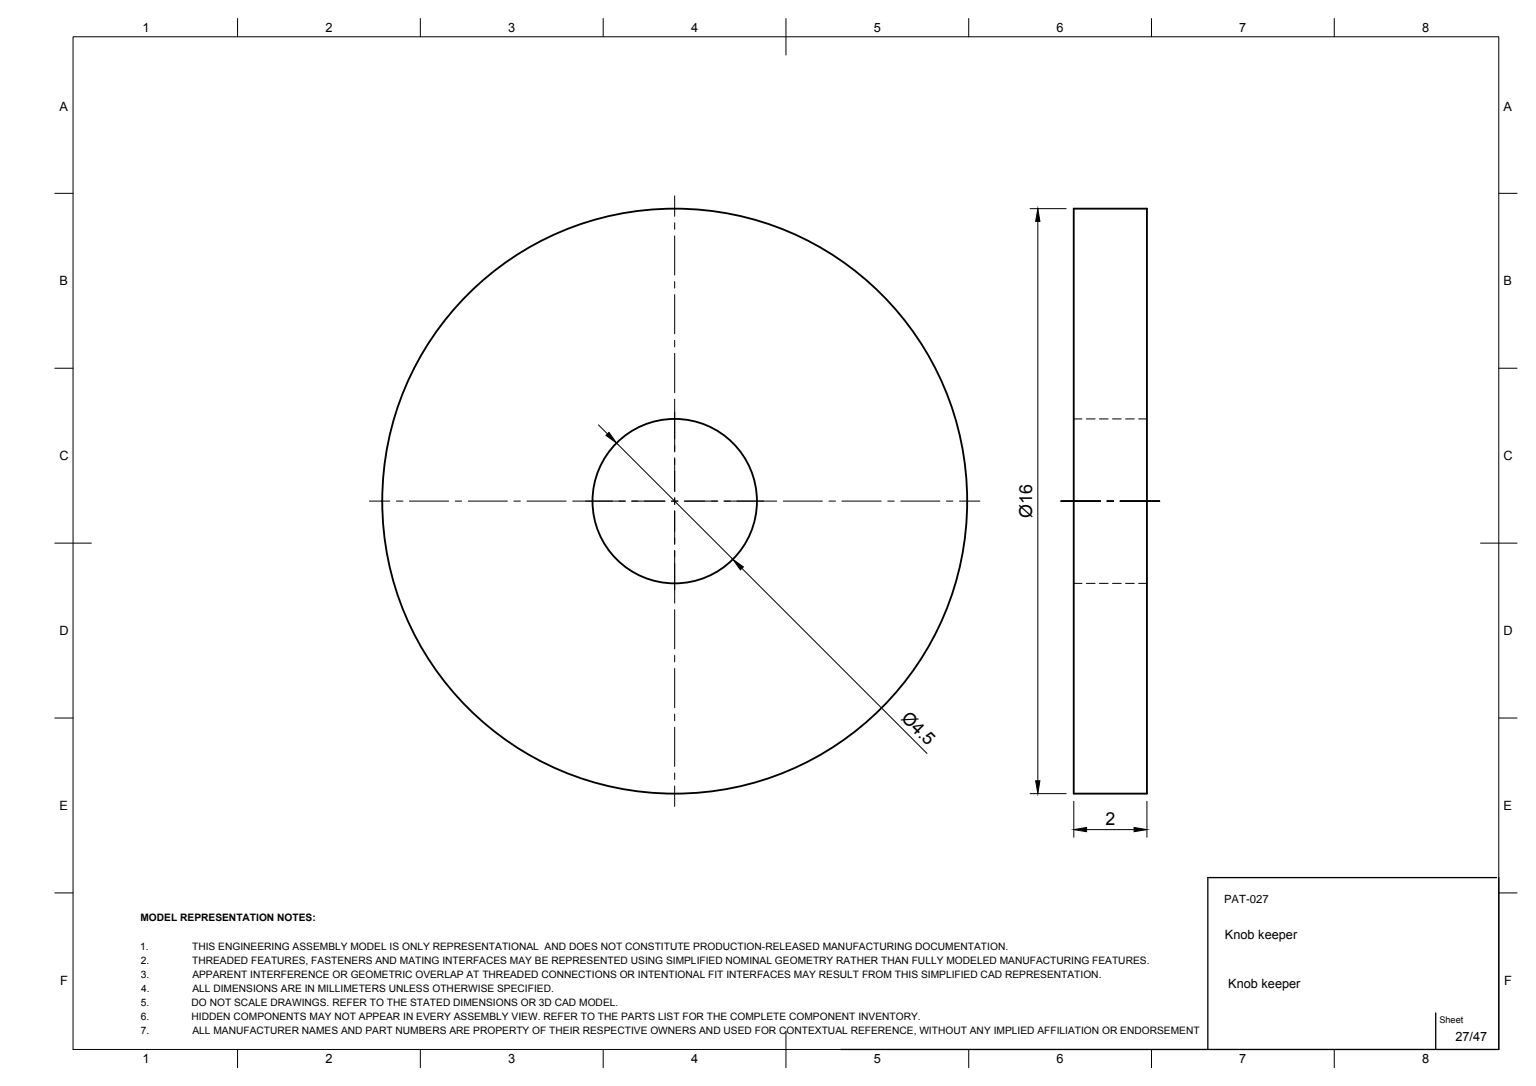
ISO-10303-21;
HEADER;
/* Generated by software containing ST-Developer
 * from STEP Tools, Inc. (www.steptools.com) 
 */

FILE_DESCRIPTION(
/* description */ ('Crank-driven oscillating fan base (mechanism only)'),

/* implementation_level */ '2;1');

FILE_NAME(
/* name */ 'Knob keeper.step',
/* time_stamp */ '2026-10-28T03:25:00-07:00',
/* author */ (''),
/* organization */ (''),
/* preprocessor_version */ 'ST-DEVELOPER v20.2',
/* originating_system */ 'Autodesk Translation Framework v15.17.0.0',
/* authorisation */ '');

FILE_SCHEMA (('AUTOMOTIVE_DESIGN { 1 0 10303 214 3 1 1 }'));
ENDSEC;

DATA;
#10=MECHANICAL_DESIGN_GEOMETRIC_PRESENTATION_REPRESENTATION('',(#464),#11916);
#376=SHAPE_REPRESENTATION_RELATIONSHIP('SRR','None',#12102,#416);
#416=ADVANCED_BREP_SHAPE_REPRESENTATION('',(#511),#11893);
#464=STYLED_ITEM('',(#12361),#511);
#511=MANIFOLD_SOLID_BREP('Body1',#6095);
#634=FACE_BOUND('',#1580,.T.);
#635=FACE_BOUND('',#1582,.T.);
#790=PLANE('',#7047);
#791=PLANE('',#7048);
#1098=FACE_OUTER_BOUND('',#1577,.T.);
#1099=FACE_OUTER_BOUND('',#1578,.T.);
#1100=FACE_OUTER_BOUND('',#1579,.T.);
#1101=FACE_OUTER_BOUND('',#1581,.T.);
#1577=EDGE_LOOP('',(#4958,#4959,#4960,#4961));
#1578=EDGE_LOOP('',(#4962,#4963,#4964,#4965));
#1579=EDGE_LOOP('',(#4966));
#1580=EDGE_LOOP('',(#4967));
#1581=EDGE_LOOP('',(#4968));
#1582=EDGE_LOOP('',(#4969));
#1966=LINE('',#11033,#2299);
#1967=LINE('',#11039,#2300);
#2299=VECTOR('',#8547,0.225);
#2300=VECTOR('',#8554,0.8);
#2705=CIRCLE('',#7042,0.225);
#2706=CIRCLE('',#7043,0.225);
#2707=CIRCLE('',#7045,0.8);
#2708=CIRCLE('',#7046,0.8);
#3136=VERTEX_POINT('',#11030);
#3137=VERTEX_POINT('',#11032);
#3138=VERTEX_POINT('',#11036);
#3139=VERTEX_POINT('',#11038);
#3774=EDGE_CURVE('',#3136,#3136,#2705,.T.);
#3775=EDGE_CURVE('',#3136,#3137,#1966,.T.);
#3776=EDGE_CURVE('',#3137,#3137,#2706,.T.);
#3777=EDGE_CURVE('',#3138,#3138,#2707,.T.);
#3778=EDGE_CURVE('',#3138,#3139,#1967,.T.);
#3779=EDGE_CURVE('',#3139,#3139,#2708,.T.);
#4958=ORIENTED_EDGE('',*,*,#3774,.F.);
#4959=ORIENTED_EDGE('',*,*,#3775,.T.);
#4960=ORIENTED_EDGE('',*,*,#3776,.T.);
#4961=ORIENTED_EDGE('',*,*,#3775,.F.);
#4962=ORIENTED_EDGE('',*,*,#3777,.F.);
#4963=ORIENTED_EDGE('',*,*,#3778,.T.);
#4964=ORIENTED_EDGE('',*,*,#3779,.T.);
#4965=ORIENTED_EDGE('',*,*,#3778,.F.);
#4966=ORIENTED_EDGE('',*,*,#3777,.T.);
#4967=ORIENTED_EDGE('',*,*,#3774,.T.);
#4968=ORIENTED_EDGE('',*,*,#3779,.F.);
#4969=ORIENTED_EDGE('',*,*,#3776,.F.);
#5635=CYLINDRICAL_SURFACE('',#7041,0.225);
#5636=CYLINDRICAL_SURFACE('',#7044,0.8);
#5904=ADVANCED_FACE('',(#1098),#5635,.F.);
#5905=ADVANCED_FACE('',(#1099),#5636,.T.);
#5906=ADVANCED_FACE('',(#1100,#634),#790,.T.);
#5907=ADVANCED_FACE('',(#1101,#635),#791,.F.);
#6095=CLOSED_SHELL('',(#5904,#5905,#5906,#5907));
#7040=AXIS2_PLACEMENT_3D('',#11028,#8541,#8542);
#7041=AXIS2_PLACEMENT_3D('',#11029,#8543,#8544);
#7042=AXIS2_PLACEMENT_3D('',#11031,#8545,#8546);
#7043=AXIS2_PLACEMENT_3D('',#11034,#8548,#8549);
#7044=AXIS2_PLACEMENT_3D('',#11035,#8550,#8551);
#7045=AXIS2_PLACEMENT_3D('',#11037,#8552,#8553);
#7046=AXIS2_PLACEMENT_3D('',#11040,#8555,#8556);
#7047=AXIS2_PLACEMENT_3D('',#11041,#8557,#8558);
#7048=AXIS2_PLACEMENT_3D('',#11042,#8559,#8560);
#8541=DIRECTION('axis',(0.,0.,1.));
#8542=DIRECTION('refdir',(1.,0.,0.));
#8543=DIRECTION('center_axis',(0.,0.,1.));
#8544=DIRECTION('ref_axis',(1.,0.,0.));
#8545=DIRECTION('center_axis',(0.,0.,-1.));
#8546=DIRECTION('ref_axis',(1.,0.,0.));
#8547=DIRECTION('',(0.,0.,-1.));
#8548=DIRECTION('center_axis',(0.,0.,-1.));
#8549=DIRECTION('ref_axis',(1.,0.,0.));
#8550=DIRECTION('center_axis',(0.,0.,1.));
#8551=DIRECTION('ref_axis',(1.,0.,0.));
#8552=DIRECTION('center_axis',(0.,0.,1.));
#8553=DIRECTION('ref_axis',(1.,0.,0.));
#8554=DIRECTION('',(0.,0.,-1.));
#8555=DIRECTION('center_axis',(0.,0.,1.));
#8556=DIRECTION('ref_axis',(1.,0.,0.));
#8557=DIRECTION('center_axis',(0.,0.,1.));
#8558=DIRECTION('ref_axis',(1.,0.,0.));
#8559=DIRECTION('center_axis',(0.,0.,1.));
#8560=DIRECTION('ref_axis',(1.,0.,0.));
#11028=CARTESIAN_POINT('',(0.,0.,0.));
#11029=CARTESIAN_POINT('Origin',(0.,0.,8.));
#11030=CARTESIAN_POINT('',(-0.225,-2.75545529808154E-17,8.2));
#11031=CARTESIAN_POINT('Origin',(0.,0.,8.2));
#11032=CARTESIAN_POINT('',(-0.225,-2.75545529808154E-17,8.));
#11033=CARTESIAN_POINT('',(-0.225,-2.75545529808154E-17,8.));
#11034=CARTESIAN_POINT('Origin',(0.,0.,8.));
#11035=CARTESIAN_POINT('Origin',(0.,0.,8.));
#11036=CARTESIAN_POINT('',(-0.8,-9.79717439317883E-17,8.2));
#11037=CARTESIAN_POINT('Origin',(0.,0.,8.2));
#11038=CARTESIAN_POINT('',(-0.8,-9.79717439317883E-17,8.));
#11039=CARTESIAN_POINT('',(-0.8,-9.79717439317883E-17,8.));
#11040=CARTESIAN_POINT('Origin',(0.,0.,8.));
#11041=CARTESIAN_POINT('Origin',(0.,0.,8.2));
#11042=CARTESIAN_POINT('Origin',(0.,0.,8.));
#11846=UNCERTAINTY_MEASURE_WITH_UNIT(LENGTH_MEASURE(0.001),#11917,
'DISTANCE_ACCURACY_VALUE',
'Maximum model space distance between geometric entities at asserted c
onnectivities');
#11869=UNCERTAINTY_MEASURE_WITH_UNIT(LENGTH_MEASURE(0.001),#11917,
'DISTANCE_ACCURACY_VALUE',
'Maximum model space distance between geometric entities at asserted c
onnectivities');
#11893=(
GEOMETRIC_REPRESENTATION_CONTEXT(3)
GLOBAL_UNCERTAINTY_ASSIGNED_CONTEXT((#11846))
GLOBAL_UNIT_ASSIGNED_CONTEXT((#11917,#11919,#11920))
REPRESENTATION_CONTEXT('','3D')
);
#11916=(
GEOMETRIC_REPRESENTATION_CONTEXT(3)
GLOBAL_UNCERTAINTY_ASSIGNED_CONTEXT((#11869))
GLOBAL_UNIT_ASSIGNED_CONTEXT((#11917,#11919,#11920))
REPRESENTATION_CONTEXT('','3D')
);
#11917=(
LENGTH_UNIT()
NAMED_UNIT(*)
SI_UNIT(.CENTI.,.METRE.)
);
#11919=(
NAMED_UNIT(*)
PLANE_ANGLE_UNIT()
SI_UNIT($,.RADIAN.)
);
#11920=(
NAMED_UNIT(*)
SI_UNIT($,.STERADIAN.)
SOLID_ANGLE_UNIT()
);
#11944=SHAPE_DEFINITION_REPRESENTATION(#11995,#12102);
#11995=PRODUCT_DEFINITION_SHAPE('',$,#12149);
#12102=SHAPE_REPRESENTATION('',(#7040),#11893);
#12125=PRODUCT_DEFINITION_CONTEXT('part definition',#12265,'design');
#12149=PRODUCT_DEFINITION('Knob keeper','Knob keeper',#12195,#12125);
#12195=PRODUCT_DEFINITION_FORMATION('',$,#12290);
#12265=APPLICATION_CONTEXT(
'Core Data for Automotive Mechanical Design Process');
#12266=PRODUCT_CONTEXT('part definition',#12265,'mechanical');
#12290=PRODUCT('Knob keeper','Knob keeper','Knob keeper',(#12266));
#12355=COLOUR_RGB('Light Blue',0.38,0.62,0.78);
#12356=FILL_AREA_STYLE_COLOUR('',#12355);
#12357=FILL_AREA_STYLE('',(#12356));
#12358=SURFACE_STYLE_FILL_AREA(#12357);
#12359=SURFACE_SIDE_STYLE('',(#12358));
#12360=SURFACE_STYLE_USAGE(.BOTH.,#12359);
#12361=PRESENTATION_STYLE_ASSIGNMENT((#12360));
ENDSEC;
END-ISO-10303-21;
